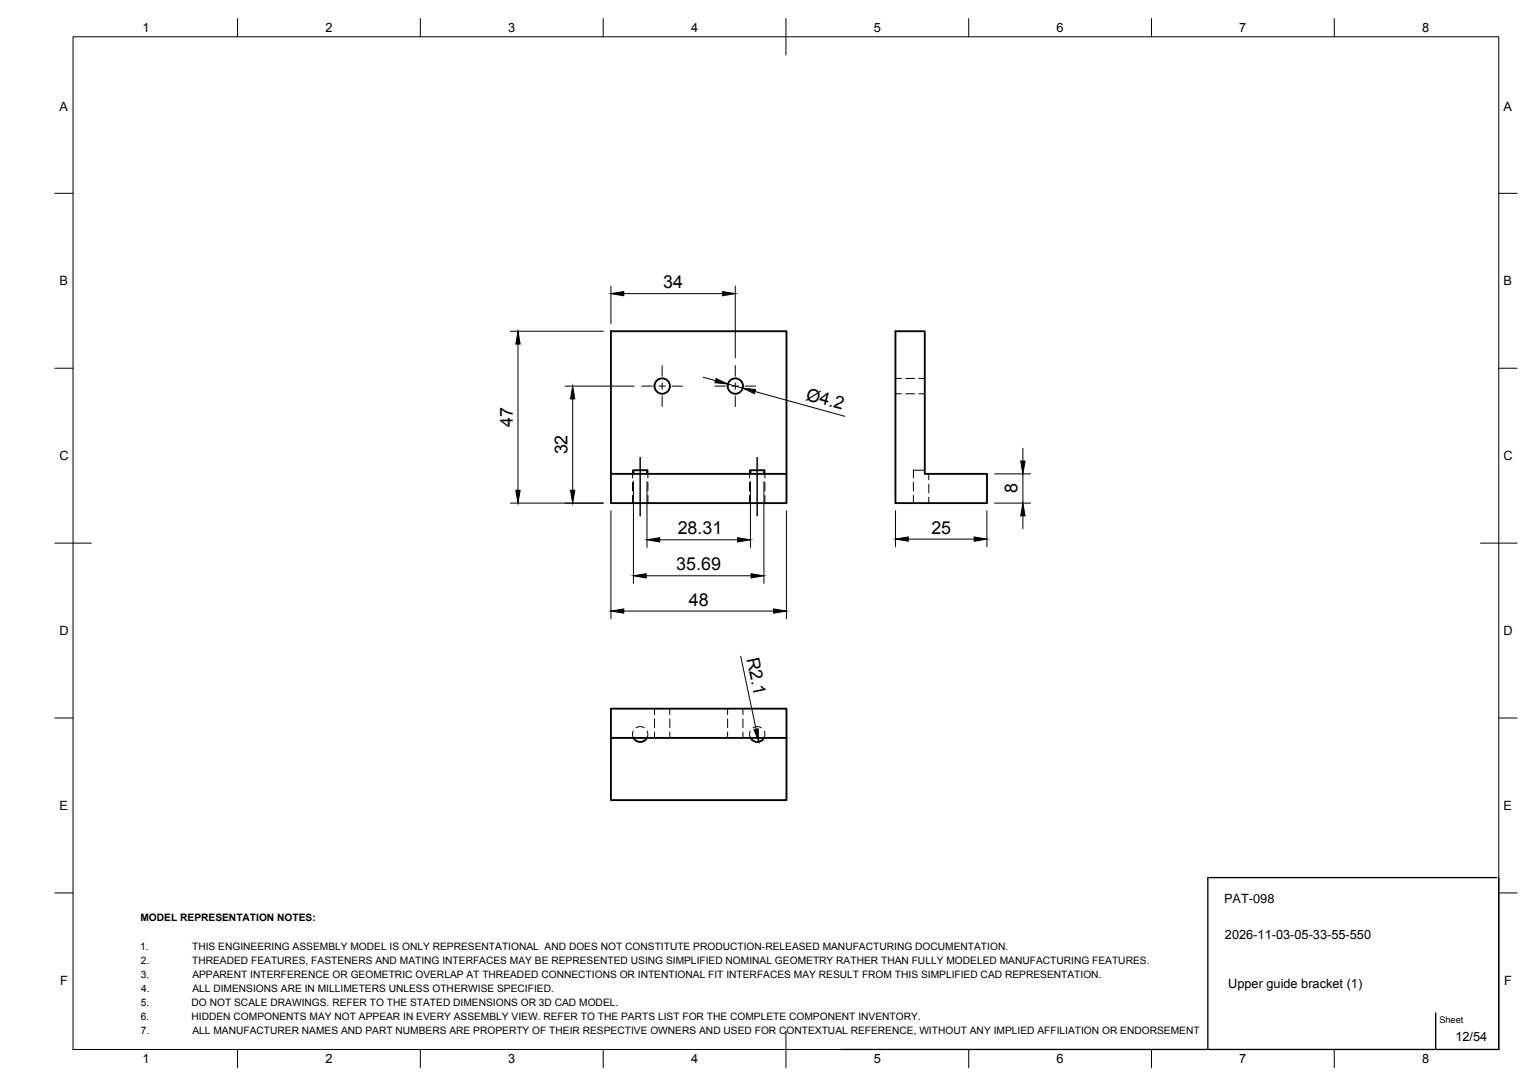
ISO-10303-21;
HEADER;
/* Generated by software containing ST-Developer
 * from STEP Tools, Inc. (www.steptools.com) 
 */

FILE_DESCRIPTION(
/* description */ ('Spring compression tester'),
/* implementation_level */ '2;1');

FILE_NAME(
/* name */ 'Upper guide bracket (1).step',
/* time_stamp */ '2026-10-28T03:24:11-07:00',
/* author */ (''),
/* organization */ (''),
/* preprocessor_version */ 'ST-DEVELOPER v20.2',
/* originating_system */ 'Autodesk Translation Framework v15.17.0.0',
/* authorisation */ '');

FILE_SCHEMA (('AUTOMOTIVE_DESIGN { 1 0 10303 214 3 1 1 }'));
ENDSEC;

DATA;
#10=MECHANICAL_DESIGN_GEOMETRIC_PRESENTATION_REPRESENTATION('',(#1113),#43521);
#993=SHAPE_REPRESENTATION_RELATIONSHIP('SRR','None',#43805,#1053);
#1053=ADVANCED_BREP_SHAPE_REPRESENTATION('',(#1188),#43465);
#1113=STYLED_ITEM('',(#44181),#1188);
#1188=MANIFOLD_SOLID_BREP('Body1',#18550);
#1339=FACE_BOUND('',#3453,.T.);
#1340=FACE_BOUND('',#3454,.T.);
#1341=FACE_BOUND('',#3458,.T.);
#1342=FACE_BOUND('',#3459,.T.);
#1343=FACE_BOUND('',#3462,.T.);
#1344=FACE_BOUND('',#3463,.T.);
#1671=PLANE('',#19555);
#1672=PLANE('',#19561);
#1673=PLANE('',#19562);
#1674=PLANE('',#19563);
#1675=PLANE('',#19564);
#1676=PLANE('',#19565);
#1677=PLANE('',#19566);
#1678=PLANE('',#19567);
#1679=PLANE('',#19568);
#1680=PLANE('',#19569);
#2306=FACE_OUTER_BOUND('',#3445,.T.);
#2307=FACE_OUTER_BOUND('',#3446,.T.);
#2308=FACE_OUTER_BOUND('',#3447,.T.);
#2309=FACE_OUTER_BOUND('',#3448,.T.);
#2310=FACE_OUTER_BOUND('',#3449,.T.);
#2311=FACE_OUTER_BOUND('',#3450,.T.);
#2312=FACE_OUTER_BOUND('',#3451,.T.);
#2313=FACE_OUTER_BOUND('',#3452,.T.);
#2314=FACE_OUTER_BOUND('',#3455,.T.);
#2315=FACE_OUTER_BOUND('',#3456,.T.);
#2316=FACE_OUTER_BOUND('',#3457,.T.);
#2317=FACE_OUTER_BOUND('',#3460,.T.);
#2318=FACE_OUTER_BOUND('',#3461,.T.);
#2319=FACE_OUTER_BOUND('',#3464,.T.);
#3445=EDGE_LOOP('',(#12841,#12842,#12843,#12844));
#3446=EDGE_LOOP('',(#12845,#12846,#12847,#12848));
#3447=EDGE_LOOP('',(#12849,#12850,#12851,#12852,#12853,#12854,#12855,#12856));
#3448=EDGE_LOOP('',(#12857,#12858,#12859));
#3449=EDGE_LOOP('',(#12860,#12861,#12862,#12863,#12864,#12865,#12866,#12867));
#3450=EDGE_LOOP('',(#12868,#12869,#12870));
#3451=EDGE_LOOP('',(#12871,#12872,#12873,#12874,#12875,#12876,#12877,#12878));
#3452=EDGE_LOOP('',(#12879,#12880,#12881,#12882,#12883,#12884,#12885,#12886,
#12887,#12888,#12889,#12890));
#3453=EDGE_LOOP('',(#12891));
#3454=EDGE_LOOP('',(#12892));
#3455=EDGE_LOOP('',(#12893,#12894,#12895,#12896));
#3456=EDGE_LOOP('',(#12897,#12898,#12899,#12900,#12901,#12902));
#3457=EDGE_LOOP('',(#12903,#12904,#12905,#12906));
#3458=EDGE_LOOP('',(#12907));
#3459=EDGE_LOOP('',(#12908));
#3460=EDGE_LOOP('',(#12909,#12910,#12911,#12912,#12913,#12914));
#3461=EDGE_LOOP('',(#12915,#12916,#12917,#12918));
#3462=EDGE_LOOP('',(#12919));
#3463=EDGE_LOOP('',(#12920));
#3464=EDGE_LOOP('',(#12921,#12922,#12923,#12924));
#4806=LINE('',#27124,#6238);
#4807=LINE('',#27130,#6239);
#4808=LINE('',#27136,#6240);
#4809=LINE('',#27140,#6241);
#4810=LINE('',#27144,#6242);
#4811=LINE('',#27147,#6243);
#4812=LINE('',#27152,#6244);
#4813=LINE('',#27156,#6245);
#4814=LINE('',#27160,#6246);
#4815=LINE('',#27163,#6247);
#4816=LINE('',#27165,#6248);
#4817=LINE('',#27167,#6249);
#4818=LINE('',#27169,#6250);
#4819=LINE('',#27171,#6251);
#4820=LINE('',#27173,#6252);
#4821=LINE('',#27174,#6253);
#4822=LINE('',#27177,#6254);
#4823=LINE('',#27179,#6255);
#4824=LINE('',#27180,#6256);
#4825=LINE('',#27184,#6257);
#4826=LINE('',#27185,#6258);
#4827=LINE('',#27186,#6259);
#4828=LINE('',#27190,#6260);
#4829=LINE('',#27191,#6261);
#4830=LINE('',#27192,#6262);
#4831=LINE('',#27196,#6263);
#4832=LINE('',#27197,#6264);
#4833=LINE('',#27198,#6265);
#4834=LINE('',#27200,#6266);
#4835=LINE('',#27201,#6267);
#6238=VECTOR('',#21920,0.21);
#6239=VECTOR('',#21927,0.21);
#6240=VECTOR('',#21934,0.21);
#6241=VECTOR('',#21937,1.);
#6242=VECTOR('',#21940,1.);
#6243=VECTOR('',#21945,1.);
#6244=VECTOR('',#21950,0.21);
#6245=VECTOR('',#21953,1.);
#6246=VECTOR('',#21956,1.);
#6247=VECTOR('',#21961,1.);
#6248=VECTOR('',#21964,1.);
#6249=VECTOR('',#21965,1.);
#6250=VECTOR('',#21966,1.);
#6251=VECTOR('',#21967,1.);
#6252=VECTOR('',#21968,1.);
#6253=VECTOR('',#21969,1.);
#6254=VECTOR('',#21972,1.);
#6255=VECTOR('',#21973,1.);
#6256=VECTOR('',#21974,1.);
#6257=VECTOR('',#21977,1.);
#6258=VECTOR('',#21978,1.);
#6259=VECTOR('',#21979,1.);
#6260=VECTOR('',#21982,1.);
#6261=VECTOR('',#21983,1.);
#6262=VECTOR('',#21984,1.);
#6263=VECTOR('',#21987,1.);
#6264=VECTOR('',#21988,1.);
#6265=VECTOR('',#21989,1.);
#6266=VECTOR('',#21992,1.);
#6267=VECTOR('',#21993,1.);
#7582=CIRCLE('',#19545,0.21);
#7583=CIRCLE('',#19546,0.21);
#7584=CIRCLE('',#19548,0.21);
#7585=CIRCLE('',#19549,0.21);
#7586=CIRCLE('',#19551,0.21);
#7587=CIRCLE('',#19552,0.21);
#7588=CIRCLE('',#19553,0.21);
#7589=CIRCLE('',#19554,0.21);
#7590=CIRCLE('',#19557,0.21);
#7591=CIRCLE('',#19558,0.21);
#7592=CIRCLE('',#19559,0.21);
#7593=CIRCLE('',#19560,0.21);
#8344=VERTEX_POINT('',#27121);
#8345=VERTEX_POINT('',#27123);
#8346=VERTEX_POINT('',#27127);
#8347=VERTEX_POINT('',#27129);
#8348=VERTEX_POINT('',#27133);
#8349=VERTEX_POINT('',#27135);
#8350=VERTEX_POINT('',#27137);
#8351=VERTEX_POINT('',#27139);
#8352=VERTEX_POINT('',#27141);
#8353=VERTEX_POINT('',#27143);
#8354=VERTEX_POINT('',#27149);
#8355=VERTEX_POINT('',#27151);
#8356=VERTEX_POINT('',#27153);
#8357=VERTEX_POINT('',#27155);
#8358=VERTEX_POINT('',#27157);
#8359=VERTEX_POINT('',#27159);
#8360=VERTEX_POINT('',#27166);
#8361=VERTEX_POINT('',#27168);
#8362=VERTEX_POINT('',#27170);
#8363=VERTEX_POINT('',#27172);
#8364=VERTEX_POINT('',#27176);
#8365=VERTEX_POINT('',#27178);
#8366=VERTEX_POINT('',#27182);
#8367=VERTEX_POINT('',#27183);
#8368=VERTEX_POINT('',#27188);
#8369=VERTEX_POINT('',#27189);
#8370=VERTEX_POINT('',#27194);
#8371=VERTEX_POINT('',#27195);
#10085=EDGE_CURVE('',#8344,#8344,#7582,.T.);
#10086=EDGE_CURVE('',#8344,#8345,#4806,.T.);
#10087=EDGE_CURVE('',#8345,#8345,#7583,.T.);
#10088=EDGE_CURVE('',#8346,#8346,#7584,.T.);
#10089=EDGE_CURVE('',#8346,#8347,#4807,.T.);
#10090=EDGE_CURVE('',#8347,#8347,#7585,.T.);
#10091=EDGE_CURVE('',#8348,#8348,#7586,.T.);
#10092=EDGE_CURVE('',#8348,#8349,#4808,.T.);
#10093=EDGE_CURVE('',#8349,#8350,#7587,.T.);
#10094=EDGE_CURVE('',#8351,#8350,#4809,.T.);
#10095=EDGE_CURVE('',#8352,#8351,#7588,.T.);
#10096=EDGE_CURVE('',#8353,#8352,#4810,.T.);
#10097=EDGE_CURVE('',#8353,#8349,#7589,.T.);
#10098=EDGE_CURVE('',#8350,#8353,#4811,.T.);
#10099=EDGE_CURVE('',#8354,#8354,#7590,.T.);
#10100=EDGE_CURVE('',#8354,#8355,#4812,.T.);
#10101=EDGE_CURVE('',#8355,#8356,#7591,.T.);
#10102=EDGE_CURVE('',#8357,#8356,#4813,.T.);
#10103=EDGE_CURVE('',#8358,#8357,#7592,.T.);
#10104=EDGE_CURVE('',#8359,#8358,#4814,.T.);
#10105=EDGE_CURVE('',#8359,#8355,#7593,.T.);
#10106=EDGE_CURVE('',#8356,#8359,#4815,.T.);
#10107=EDGE_CURVE('',#8351,#8358,#4816,.T.);
#10108=EDGE_CURVE('',#8357,#8360,#4817,.T.);
#10109=EDGE_CURVE('',#8361,#8360,#4818,.T.);
#10110=EDGE_CURVE('',#8361,#8362,#4819,.T.);
#10111=EDGE_CURVE('',#8362,#8363,#4820,.T.);
#10112=EDGE_CURVE('',#8363,#8352,#4821,.T.);
#10113=EDGE_CURVE('',#8363,#8364,#4822,.T.);
#10114=EDGE_CURVE('',#8365,#8364,#4823,.T.);
#10115=EDGE_CURVE('',#8360,#8365,#4824,.T.);
#10116=EDGE_CURVE('',#8366,#8367,#4825,.T.);
#10117=EDGE_CURVE('',#8367,#8365,#4826,.T.);
#10118=EDGE_CURVE('',#8364,#8366,#4827,.T.);
#10119=EDGE_CURVE('',#8368,#8369,#4828,.T.);
#10120=EDGE_CURVE('',#8368,#8361,#4829,.T.);
#10121=EDGE_CURVE('',#8369,#8367,#4830,.T.);
#10122=EDGE_CURVE('',#8370,#8371,#4831,.T.);
#10123=EDGE_CURVE('',#8370,#8368,#4832,.T.);
#10124=EDGE_CURVE('',#8371,#8369,#4833,.T.);
#10125=EDGE_CURVE('',#8362,#8370,#4834,.T.);
#10126=EDGE_CURVE('',#8371,#8366,#4835,.T.);
#12841=ORIENTED_EDGE('',*,*,#10085,.F.);
#12842=ORIENTED_EDGE('',*,*,#10086,.T.);
#12843=ORIENTED_EDGE('',*,*,#10087,.F.);
#12844=ORIENTED_EDGE('',*,*,#10086,.F.);
#12845=ORIENTED_EDGE('',*,*,#10088,.F.);
#12846=ORIENTED_EDGE('',*,*,#10089,.T.);
#12847=ORIENTED_EDGE('',*,*,#10090,.F.);
#12848=ORIENTED_EDGE('',*,*,#10089,.F.);
#12849=ORIENTED_EDGE('',*,*,#10091,.F.);
#12850=ORIENTED_EDGE('',*,*,#10092,.T.);
#12851=ORIENTED_EDGE('',*,*,#10093,.T.);
#12852=ORIENTED_EDGE('',*,*,#10094,.F.);
#12853=ORIENTED_EDGE('',*,*,#10095,.F.);
#12854=ORIENTED_EDGE('',*,*,#10096,.F.);
#12855=ORIENTED_EDGE('',*,*,#10097,.T.);
#12856=ORIENTED_EDGE('',*,*,#10092,.F.);
#12857=ORIENTED_EDGE('',*,*,#10098,.F.);
#12858=ORIENTED_EDGE('',*,*,#10093,.F.);
#12859=ORIENTED_EDGE('',*,*,#10097,.F.);
#12860=ORIENTED_EDGE('',*,*,#10099,.F.);
#12861=ORIENTED_EDGE('',*,*,#10100,.T.);
#12862=ORIENTED_EDGE('',*,*,#10101,.T.);
#12863=ORIENTED_EDGE('',*,*,#10102,.F.);
#12864=ORIENTED_EDGE('',*,*,#10103,.F.);
#12865=ORIENTED_EDGE('',*,*,#10104,.F.);
#12866=ORIENTED_EDGE('',*,*,#10105,.T.);
#12867=ORIENTED_EDGE('',*,*,#10100,.F.);
#12868=ORIENTED_EDGE('',*,*,#10106,.F.);
#12869=ORIENTED_EDGE('',*,*,#10101,.F.);
#12870=ORIENTED_EDGE('',*,*,#10105,.F.);
#12871=ORIENTED_EDGE('',*,*,#10095,.T.);
#12872=ORIENTED_EDGE('',*,*,#10107,.T.);
#12873=ORIENTED_EDGE('',*,*,#10103,.T.);
#12874=ORIENTED_EDGE('',*,*,#10108,.T.);
#12875=ORIENTED_EDGE('',*,*,#10109,.F.);
#12876=ORIENTED_EDGE('',*,*,#10110,.T.);
#12877=ORIENTED_EDGE('',*,*,#10111,.T.);
#12878=ORIENTED_EDGE('',*,*,#10112,.T.);
#12879=ORIENTED_EDGE('',*,*,#10096,.T.);
#12880=ORIENTED_EDGE('',*,*,#10112,.F.);
#12881=ORIENTED_EDGE('',*,*,#10113,.T.);
#12882=ORIENTED_EDGE('',*,*,#10114,.F.);
#12883=ORIENTED_EDGE('',*,*,#10115,.F.);
#12884=ORIENTED_EDGE('',*,*,#10108,.F.);
#12885=ORIENTED_EDGE('',*,*,#10102,.T.);
#12886=ORIENTED_EDGE('',*,*,#10106,.T.);
#12887=ORIENTED_EDGE('',*,*,#10104,.T.);
#12888=ORIENTED_EDGE('',*,*,#10107,.F.);
#12889=ORIENTED_EDGE('',*,*,#10094,.T.);
#12890=ORIENTED_EDGE('',*,*,#10098,.T.);
#12891=ORIENTED_EDGE('',*,*,#10085,.T.);
#12892=ORIENTED_EDGE('',*,*,#10088,.T.);
#12893=ORIENTED_EDGE('',*,*,#10116,.T.);
#12894=ORIENTED_EDGE('',*,*,#10117,.T.);
#12895=ORIENTED_EDGE('',*,*,#10114,.T.);
#12896=ORIENTED_EDGE('',*,*,#10118,.T.);
#12897=ORIENTED_EDGE('',*,*,#10119,.F.);
#12898=ORIENTED_EDGE('',*,*,#10120,.T.);
#12899=ORIENTED_EDGE('',*,*,#10109,.T.);
#12900=ORIENTED_EDGE('',*,*,#10115,.T.);
#12901=ORIENTED_EDGE('',*,*,#10117,.F.);
#12902=ORIENTED_EDGE('',*,*,#10121,.F.);
#12903=ORIENTED_EDGE('',*,*,#10122,.F.);
#12904=ORIENTED_EDGE('',*,*,#10123,.T.);
#12905=ORIENTED_EDGE('',*,*,#10119,.T.);
#12906=ORIENTED_EDGE('',*,*,#10124,.F.);
#12907=ORIENTED_EDGE('',*,*,#10091,.T.);
#12908=ORIENTED_EDGE('',*,*,#10099,.T.);
#12909=ORIENTED_EDGE('',*,*,#10111,.F.);
#12910=ORIENTED_EDGE('',*,*,#10125,.T.);
#12911=ORIENTED_EDGE('',*,*,#10122,.T.);
#12912=ORIENTED_EDGE('',*,*,#10126,.T.);
#12913=ORIENTED_EDGE('',*,*,#10118,.F.);
#12914=ORIENTED_EDGE('',*,*,#10113,.F.);
#12915=ORIENTED_EDGE('',*,*,#10126,.F.);
#12916=ORIENTED_EDGE('',*,*,#10124,.T.);
#12917=ORIENTED_EDGE('',*,*,#10121,.T.);
#12918=ORIENTED_EDGE('',*,*,#10116,.F.);
#12919=ORIENTED_EDGE('',*,*,#10087,.T.);
#12920=ORIENTED_EDGE('',*,*,#10090,.T.);
#12921=ORIENTED_EDGE('',*,*,#10125,.F.);
#12922=ORIENTED_EDGE('',*,*,#10110,.F.);
#12923=ORIENTED_EDGE('',*,*,#10120,.F.);
#12924=ORIENTED_EDGE('',*,*,#10123,.F.);
#17159=CYLINDRICAL_SURFACE('',#19544,0.21);
#17160=CYLINDRICAL_SURFACE('',#19547,0.21);
#17161=CYLINDRICAL_SURFACE('',#19550,0.21);
#17162=CYLINDRICAL_SURFACE('',#19556,0.21);
#17630=ADVANCED_FACE('',(#2306),#17159,.F.);
#17631=ADVANCED_FACE('',(#2307),#17160,.F.);
#17632=ADVANCED_FACE('',(#2308),#17161,.F.);
#17633=ADVANCED_FACE('',(#2309),#1671,.F.);
#17634=ADVANCED_FACE('',(#2310),#17162,.F.);
#17635=ADVANCED_FACE('',(#2311),#1672,.F.);
#17636=ADVANCED_FACE('',(#2312),#1673,.T.);
#17637=ADVANCED_FACE('',(#2313,#1339,#1340),#1674,.T.);
#17638=ADVANCED_FACE('',(#2314),#1675,.T.);
#17639=ADVANCED_FACE('',(#2315),#1676,.T.);
#17640=ADVANCED_FACE('',(#2316,#1341,#1342),#1677,.T.);
#17641=ADVANCED_FACE('',(#2317),#1678,.T.);
#17642=ADVANCED_FACE('',(#2318,#1343,#1344),#1679,.T.);
#17643=ADVANCED_FACE('',(#2319),#1680,.F.);
#18550=CLOSED_SHELL('',(#17630,#17631,#17632,#17633,#17634,#17635,#17636,
#17637,#17638,#17639,#17640,#17641,#17642,#17643));
#19543=AXIS2_PLACEMENT_3D('',#27119,#21914,#21915);
#19544=AXIS2_PLACEMENT_3D('',#27120,#21916,#21917);
#19545=AXIS2_PLACEMENT_3D('',#27122,#21918,#21919);
#19546=AXIS2_PLACEMENT_3D('',#27125,#21921,#21922);
#19547=AXIS2_PLACEMENT_3D('',#27126,#21923,#21924);
#19548=AXIS2_PLACEMENT_3D('',#27128,#21925,#21926);
#19549=AXIS2_PLACEMENT_3D('',#27131,#21928,#21929);
#19550=AXIS2_PLACEMENT_3D('',#27132,#21930,#21931);
#19551=AXIS2_PLACEMENT_3D('',#27134,#21932,#21933);
#19552=AXIS2_PLACEMENT_3D('',#27138,#21935,#21936);
#19553=AXIS2_PLACEMENT_3D('',#27142,#21938,#21939);
#19554=AXIS2_PLACEMENT_3D('',#27145,#21941,#21942);
#19555=AXIS2_PLACEMENT_3D('',#27146,#21943,#21944);
#19556=AXIS2_PLACEMENT_3D('',#27148,#21946,#21947);
#19557=AXIS2_PLACEMENT_3D('',#27150,#21948,#21949);
#19558=AXIS2_PLACEMENT_3D('',#27154,#21951,#21952);
#19559=AXIS2_PLACEMENT_3D('',#27158,#21954,#21955);
#19560=AXIS2_PLACEMENT_3D('',#27161,#21957,#21958);
#19561=AXIS2_PLACEMENT_3D('',#27162,#21959,#21960);
#19562=AXIS2_PLACEMENT_3D('',#27164,#21962,#21963);
#19563=AXIS2_PLACEMENT_3D('',#27175,#21970,#21971);
#19564=AXIS2_PLACEMENT_3D('',#27181,#21975,#21976);
#19565=AXIS2_PLACEMENT_3D('',#27187,#21980,#21981);
#19566=AXIS2_PLACEMENT_3D('',#27193,#21985,#21986);
#19567=AXIS2_PLACEMENT_3D('',#27199,#21990,#21991);
#19568=AXIS2_PLACEMENT_3D('',#27202,#21994,#21995);
#19569=AXIS2_PLACEMENT_3D('',#27203,#21996,#21997);
#21914=DIRECTION('axis',(0.,0.,1.));
#21915=DIRECTION('refdir',(1.,0.,0.));
#21916=DIRECTION('center_axis',(0.,0.,1.));
#21917=DIRECTION('ref_axis',(1.,0.,0.));
#21918=DIRECTION('center_axis',(0.,0.,1.));
#21919=DIRECTION('ref_axis',(1.,0.,0.));
#21920=DIRECTION('',(0.,0.,1.));
#21921=DIRECTION('center_axis',(0.,0.,-1.));
#21922=DIRECTION('ref_axis',(1.,0.,0.));
#21923=DIRECTION('center_axis',(0.,0.,1.));
#21924=DIRECTION('ref_axis',(1.,0.,0.));
#21925=DIRECTION('center_axis',(0.,0.,1.));
#21926=DIRECTION('ref_axis',(1.,0.,0.));
#21927=DIRECTION('',(0.,0.,1.));
#21928=DIRECTION('center_axis',(0.,0.,-1.));
#21929=DIRECTION('ref_axis',(1.,0.,0.));
#21930=DIRECTION('center_axis',(0.,1.,0.));
#21931=DIRECTION('ref_axis',(1.,0.,0.));
#21932=DIRECTION('center_axis',(0.,1.,0.));
#21933=DIRECTION('ref_axis',(1.,0.,0.));
#21934=DIRECTION('',(0.,1.,0.));
#21935=DIRECTION('center_axis',(0.,1.,0.));
#21936=DIRECTION('ref_axis',(1.,0.,0.));
#21937=DIRECTION('',(0.,1.,0.));
#21938=DIRECTION('center_axis',(0.,-1.,0.));
#21939=DIRECTION('ref_axis',(1.,0.,0.));
#21940=DIRECTION('',(0.,-1.,0.));
#21941=DIRECTION('center_axis',(0.,1.,0.));
#21942=DIRECTION('ref_axis',(1.,0.,0.));
#21943=DIRECTION('center_axis',(0.,1.,0.));
#21944=DIRECTION('ref_axis',(1.,0.,0.));
#21945=DIRECTION('',(-1.,0.,0.));
#21946=DIRECTION('center_axis',(0.,1.,0.));
#21947=DIRECTION('ref_axis',(1.,0.,0.));
#21948=DIRECTION('center_axis',(0.,1.,0.));
#21949=DIRECTION('ref_axis',(1.,0.,0.));
#21950=DIRECTION('',(0.,1.,0.));
#21951=DIRECTION('center_axis',(0.,1.,0.));
#21952=DIRECTION('ref_axis',(1.,0.,0.));
#21953=DIRECTION('',(0.,1.,0.));
#21954=DIRECTION('center_axis',(0.,-1.,0.));
#21955=DIRECTION('ref_axis',(1.,0.,0.));
#21956=DIRECTION('',(0.,-1.,0.));
#21957=DIRECTION('center_axis',(0.,1.,0.));
#21958=DIRECTION('ref_axis',(1.,0.,0.));
#21959=DIRECTION('center_axis',(0.,1.,0.));
#21960=DIRECTION('ref_axis',(1.,0.,0.));
#21961=DIRECTION('',(-1.,0.,0.));
#21962=DIRECTION('center_axis',(0.,1.,0.));
#21963=DIRECTION('ref_axis',(-1.,0.,0.));
#21964=DIRECTION('',(1.,0.,0.));
#21965=DIRECTION('',(1.,0.,0.));
#21966=DIRECTION('',(0.,0.,1.));
#21967=DIRECTION('',(-1.,0.,0.));
#21968=DIRECTION('',(0.,0.,1.));
#21969=DIRECTION('',(1.,0.,0.));
#21970=DIRECTION('center_axis',(0.,0.,-1.));
#21971=DIRECTION('ref_axis',(-1.,0.,0.));
#21972=DIRECTION('',(0.,1.,0.));
#21973=DIRECTION('',(-1.,0.,0.));
#21974=DIRECTION('',(0.,1.,0.));
#21975=DIRECTION('center_axis',(0.,1.,0.));
#21976=DIRECTION('ref_axis',(0.,0.,1.));
#21977=DIRECTION('',(1.,0.,0.));
#21978=DIRECTION('',(0.,0.,-1.));
#21979=DIRECTION('',(0.,0.,1.));
#21980=DIRECTION('center_axis',(1.,0.,0.));
#21981=DIRECTION('ref_axis',(0.,1.,0.));
#21982=DIRECTION('',(0.,0.,1.));
#21983=DIRECTION('',(0.,1.,0.));
#21984=DIRECTION('',(0.,1.,0.));
#21985=DIRECTION('center_axis',(0.,-1.,0.));
#21986=DIRECTION('ref_axis',(1.,0.,0.));
#21987=DIRECTION('',(0.,0.,1.));
#21988=DIRECTION('',(1.,0.,0.));
#21989=DIRECTION('',(1.,0.,0.));
#21990=DIRECTION('center_axis',(-1.,0.,0.));
#21991=DIRECTION('ref_axis',(0.,-1.,0.));
#21992=DIRECTION('',(0.,-1.,0.));
#21993=DIRECTION('',(0.,1.,0.));
#21994=DIRECTION('center_axis',(0.,0.,1.));
#21995=DIRECTION('ref_axis',(1.,0.,0.));
#21996=DIRECTION('center_axis',(0.,0.,1.));
#21997=DIRECTION('ref_axis',(1.,0.,0.));
#27119=CARTESIAN_POINT('',(0.,0.,0.));
#27120=CARTESIAN_POINT('Origin',(5.,5.5,29.6));
#27121=CARTESIAN_POINT('',(4.79,5.5,29.7));
#27122=CARTESIAN_POINT('Origin',(5.,5.5,29.7));
#27123=CARTESIAN_POINT('',(4.79,5.5,30.5));
#27124=CARTESIAN_POINT('',(4.79,5.5,29.6));
#27125=CARTESIAN_POINT('Origin',(5.,5.5,30.5));
#27126=CARTESIAN_POINT('Origin',(7.,5.5,29.6));
#27127=CARTESIAN_POINT('',(6.79,5.5,29.7));
#27128=CARTESIAN_POINT('Origin',(7.,5.5,29.7));
#27129=CARTESIAN_POINT('',(6.79,5.5,30.5));
#27130=CARTESIAN_POINT('',(6.79,5.5,29.6));
#27131=CARTESIAN_POINT('Origin',(7.,5.5,30.5));
#27132=CARTESIAN_POINT('Origin',(4.4,2.2,29.8));
#27133=CARTESIAN_POINT('',(4.19,2.3,29.8));
#27134=CARTESIAN_POINT('Origin',(4.4,2.3,29.8));
#27135=CARTESIAN_POINT('',(4.19,3.2,29.8));
#27136=CARTESIAN_POINT('',(4.19,2.2,29.8));
#27137=CARTESIAN_POINT('',(4.58466185312619,3.2,29.7));
#27138=CARTESIAN_POINT('Origin',(4.4,3.2,29.8));
#27139=CARTESIAN_POINT('',(4.5846618531262,3.1,29.7));
#27140=CARTESIAN_POINT('',(4.58466185312619,2.2,29.7));
#27141=CARTESIAN_POINT('',(4.21533814687381,3.1,29.7));
#27142=CARTESIAN_POINT('Origin',(4.4,3.1,29.8));
#27143=CARTESIAN_POINT('',(4.21533814687381,3.2,29.7));
#27144=CARTESIAN_POINT('',(4.21533814687381,2.2,29.7));
#27145=CARTESIAN_POINT('Origin',(4.4,3.2,29.8));
#27146=CARTESIAN_POINT('Origin',(4.4,3.2,29.8));
#27147=CARTESIAN_POINT('',(6.4,3.2,29.7));
#27148=CARTESIAN_POINT('Origin',(7.6,2.2,29.8));
#27149=CARTESIAN_POINT('',(7.39,2.3,29.8));
#27150=CARTESIAN_POINT('Origin',(7.6,2.3,29.8));
#27151=CARTESIAN_POINT('',(7.39,3.2,29.8));
#27152=CARTESIAN_POINT('',(7.39,2.2,29.8));
#27153=CARTESIAN_POINT('',(7.78466185312619,3.2,29.7));
#27154=CARTESIAN_POINT('Origin',(7.6,3.2,29.8));
#27155=CARTESIAN_POINT('',(7.78466185312619,3.1,29.7));
#27156=CARTESIAN_POINT('',(7.78466185312619,2.2,29.7));
#27157=CARTESIAN_POINT('',(7.4153381468738,3.1,29.7));
#27158=CARTESIAN_POINT('Origin',(7.6,3.1,29.8));
#27159=CARTESIAN_POINT('',(7.41533814687381,3.2,29.7));
#27160=CARTESIAN_POINT('',(7.41533814687381,2.2,29.7));
#27161=CARTESIAN_POINT('Origin',(7.6,3.2,29.8));
#27162=CARTESIAN_POINT('Origin',(7.6,3.2,29.8));
#27163=CARTESIAN_POINT('',(8.,3.2,29.7));
#27164=CARTESIAN_POINT('Origin',(8.4,3.1,28.));
#27165=CARTESIAN_POINT('',(8.4,3.1,29.7));
#27166=CARTESIAN_POINT('',(8.4,3.1,29.7));
#27167=CARTESIAN_POINT('',(8.4,3.1,29.7));
#27168=CARTESIAN_POINT('',(8.4,3.1,28.));
#27169=CARTESIAN_POINT('',(8.4,3.1,28.));
#27170=CARTESIAN_POINT('',(3.6,3.1,28.));
#27171=CARTESIAN_POINT('',(8.4,3.1,28.));
#27172=CARTESIAN_POINT('',(3.6,3.1,29.7));
#27173=CARTESIAN_POINT('',(3.6,3.1,28.));
#27174=CARTESIAN_POINT('',(8.4,3.1,29.7));
#27175=CARTESIAN_POINT('Origin',(8.4,2.3,29.7));
#27176=CARTESIAN_POINT('',(3.6,7.,29.7));
#27177=CARTESIAN_POINT('',(3.6,2.3,29.7));
#27178=CARTESIAN_POINT('',(8.4,7.,29.7));
#27179=CARTESIAN_POINT('',(3.6,7.,29.7));
#27180=CARTESIAN_POINT('',(8.4,2.3,29.7));
#27181=CARTESIAN_POINT('Origin',(6.,7.,30.1));
#27182=CARTESIAN_POINT('',(3.6,7.,30.5));
#27183=CARTESIAN_POINT('',(8.4,7.,30.5));
#27184=CARTESIAN_POINT('',(8.4,7.,30.5));
#27185=CARTESIAN_POINT('',(8.4,7.,29.7));
#27186=CARTESIAN_POINT('',(3.6,7.,30.5));
#27187=CARTESIAN_POINT('Origin',(8.4,2.3,28.));
#27188=CARTESIAN_POINT('',(8.4,2.3,28.));
#27189=CARTESIAN_POINT('',(8.4,2.3,30.5));
#27190=CARTESIAN_POINT('',(8.4,2.3,28.));
#27191=CARTESIAN_POINT('',(8.4,2.3,28.));
#27192=CARTESIAN_POINT('',(8.4,2.3,30.5));
#27193=CARTESIAN_POINT('Origin',(3.6,2.3,28.));
#27194=CARTESIAN_POINT('',(3.6,2.3,28.));
#27195=CARTESIAN_POINT('',(3.6,2.3,30.5));
#27196=CARTESIAN_POINT('',(3.6,2.3,28.));
#27197=CARTESIAN_POINT('',(3.6,2.3,28.));
#27198=CARTESIAN_POINT('',(3.6,2.3,30.5));
#27199=CARTESIAN_POINT('Origin',(3.6,3.1,28.));
#27200=CARTESIAN_POINT('',(3.6,3.1,28.));
#27201=CARTESIAN_POINT('',(3.6,2.3,30.5));
#27202=CARTESIAN_POINT('Origin',(6.,2.7,30.5));
#27203=CARTESIAN_POINT('Origin',(6.,2.7,28.));
#43397=UNCERTAINTY_MEASURE_WITH_UNIT(LENGTH_MEASURE(0.001),#43522,
'DISTANCE_ACCURACY_VALUE',
'Maximum model space distance between geometric entities at asserted c
onnectivities');
#43453=UNCERTAINTY_MEASURE_WITH_UNIT(LENGTH_MEASURE(0.001),#43522,
'DISTANCE_ACCURACY_VALUE',
'Maximum model space distance between geometric entities at asserted c
onnectivities');
#43465=(
GEOMETRIC_REPRESENTATION_CONTEXT(3)
GLOBAL_UNCERTAINTY_ASSIGNED_CONTEXT((#43397))
GLOBAL_UNIT_ASSIGNED_CONTEXT((#43522,#43524,#43525))
REPRESENTATION_CONTEXT('','3D')
);
#43521=(
GEOMETRIC_REPRESENTATION_CONTEXT(3)
GLOBAL_UNCERTAINTY_ASSIGNED_CONTEXT((#43453))
GLOBAL_UNIT_ASSIGNED_CONTEXT((#43522,#43524,#43525))
REPRESENTATION_CONTEXT('','3D')
);
#43522=(
LENGTH_UNIT()
NAMED_UNIT(*)
SI_UNIT(.CENTI.,.METRE.)
);
#43524=(
NAMED_UNIT(*)
PLANE_ANGLE_UNIT()
SI_UNIT($,.RADIAN.)
);
#43525=(
NAMED_UNIT(*)
SI_UNIT($,.STERADIAN.)
SOLID_ANGLE_UNIT()
);
#43537=SHAPE_DEFINITION_REPRESENTATION(#43604,#43805);
#43604=PRODUCT_DEFINITION_SHAPE('',$,#43873);
#43805=SHAPE_REPRESENTATION('',(#19543),#43465);
#43861=PRODUCT_DEFINITION_CONTEXT('part definition',#44064,'design');
#43873=PRODUCT_DEFINITION('Upper guide bracket (1)',
'Upper guide bracket (1)',#43940,#43861);
#43940=PRODUCT_DEFINITION_FORMATION('',$,#44077);
#44064=APPLICATION_CONTEXT(
'Core Data for Automotive Mechanical Design Process');
#44065=PRODUCT_CONTEXT('part definition',#44064,'mechanical');
#44077=PRODUCT('Upper guide bracket (1)','Upper guide bracket (1)',
'Upper guide bracket (1)',(#44065));
#44175=COLOUR_RGB('Dark Blue',0.08,0.2,0.34);
#44176=FILL_AREA_STYLE_COLOUR('',#44175);
#44177=FILL_AREA_STYLE('',(#44176));
#44178=SURFACE_STYLE_FILL_AREA(#44177);
#44179=SURFACE_SIDE_STYLE('',(#44178));
#44180=SURFACE_STYLE_USAGE(.BOTH.,#44179);
#44181=PRESENTATION_STYLE_ASSIGNMENT((#44180));
ENDSEC;
END-ISO-10303-21;
